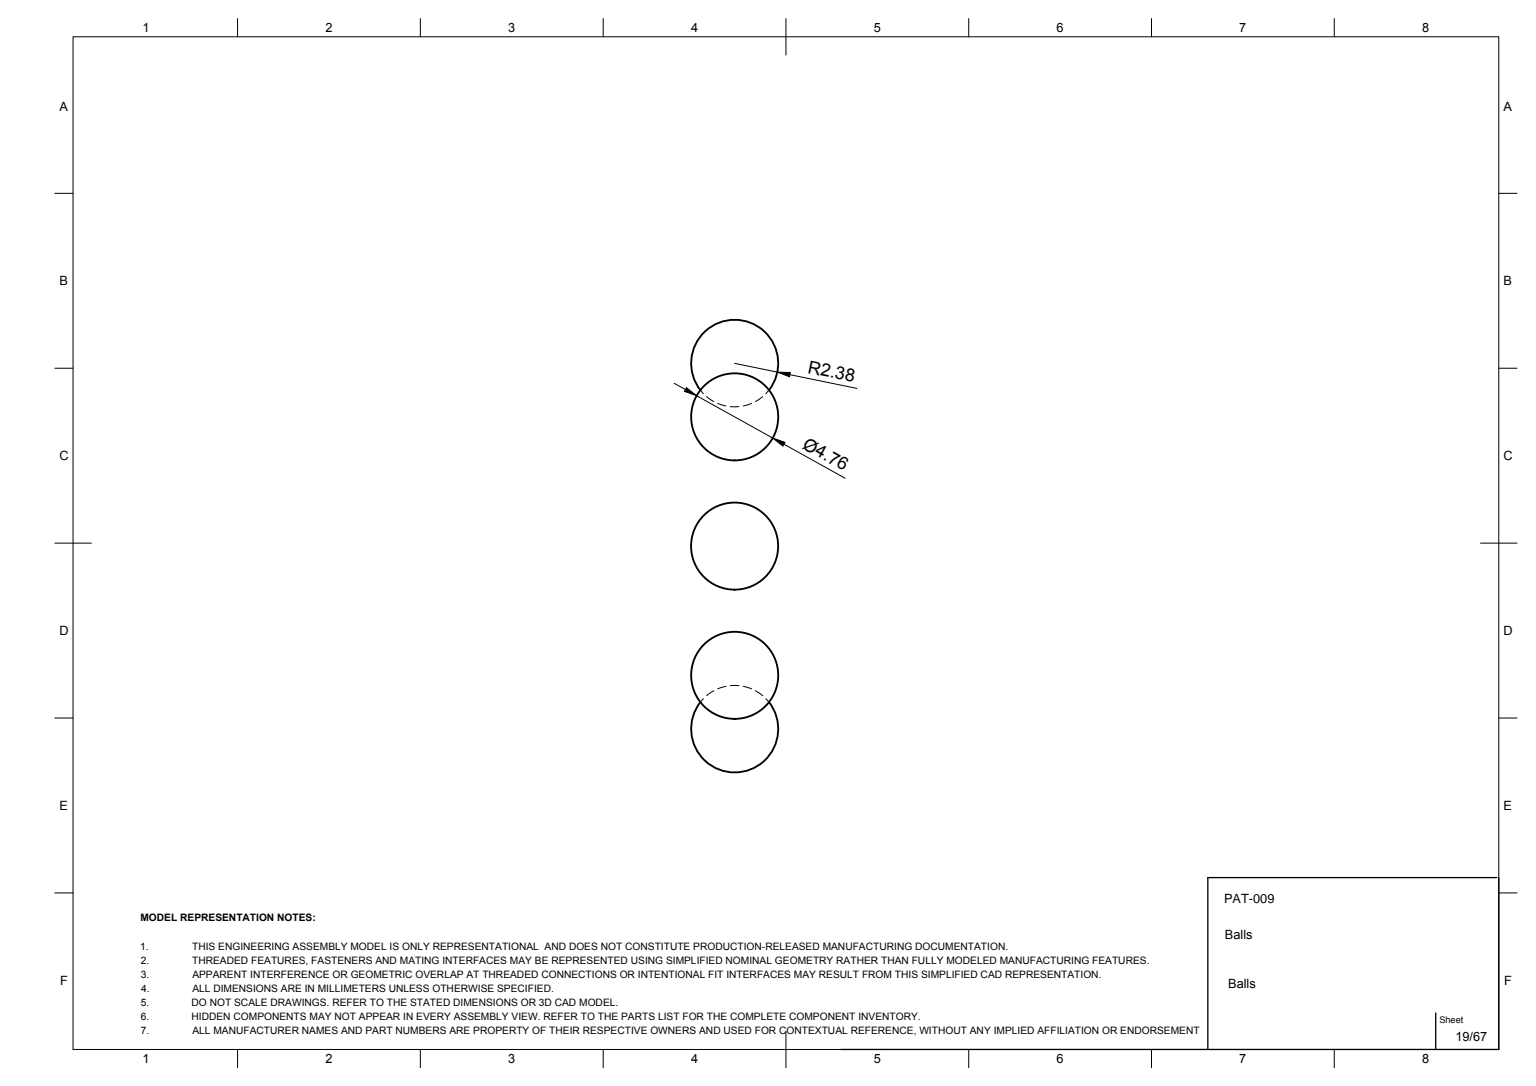
ISO-10303-21;
HEADER;
/* Generated by software containing ST-Developer
 * from STEP Tools, Inc. (www.steptools.com) 
 */

FILE_DESCRIPTION(
/* description */ ('Bell-crank linkage with push rods'),
/* implementation_level */ '2;1');

FILE_NAME(
/* name */ 'Balls.step',
/* time_stamp */ '2026-10-28T03:25:15-07:00',
/* author */ (''),
/* organization */ (''),
/* preprocessor_version */ 'ST-DEVELOPER v20.2',
/* originating_system */ 'Autodesk Translation Framework v15.17.0.0',
/* authorisation */ '');

FILE_SCHEMA (('AUTOMOTIVE_DESIGN { 1 0 10303 214 3 1 1 }'));
ENDSEC;

DATA;
#10=MECHANICAL_DESIGN_GEOMETRIC_PRESENTATION_REPRESENTATION('',(#616,#617,#618,#619,#620,#621,#622,#623),#16678);
#415=SPHERICAL_SURFACE('',#9830,0.23815);
#416=SPHERICAL_SURFACE('',#9832,0.23815);
#417=SPHERICAL_SURFACE('',#9834,0.23815);
#418=SPHERICAL_SURFACE('',#9836,0.23815);
#419=SPHERICAL_SURFACE('',#9838,0.23815);
#420=SPHERICAL_SURFACE('',#9840,0.23815);
#421=SPHERICAL_SURFACE('',#9842,0.23815);
#422=SPHERICAL_SURFACE('',#9844,0.23815);
#508=SHAPE_REPRESENTATION_RELATIONSHIP('SRR','None',#16925,#562);
#562=ADVANCED_BREP_SHAPE_REPRESENTATION('',(#677,#678,#679,#680,#681,#682,
#683,#684),#16630);
#616=STYLED_ITEM('',(#17291),#677);
#617=STYLED_ITEM('',(#17291),#678);
#618=STYLED_ITEM('',(#17291),#679);
#619=STYLED_ITEM('',(#17291),#680);
#620=STYLED_ITEM('',(#17291),#681);
#621=STYLED_ITEM('',(#17291),#682);
#622=STYLED_ITEM('',(#17291),#683);
#623=STYLED_ITEM('',(#17291),#684);
#677=MANIFOLD_SOLID_BREP('Body1',#8807);
#678=MANIFOLD_SOLID_BREP('Body2',#8808);
#679=MANIFOLD_SOLID_BREP('Body3',#8809);
#680=MANIFOLD_SOLID_BREP('Body4',#8810);
#681=MANIFOLD_SOLID_BREP('Body5',#8811);
#682=MANIFOLD_SOLID_BREP('Body6',#8812);
#683=MANIFOLD_SOLID_BREP('Body7',#8813);
#684=MANIFOLD_SOLID_BREP('Body8',#8814);
#1426=FACE_OUTER_BOUND('',#2040,.T.);
#1427=FACE_OUTER_BOUND('',#2041,.T.);
#1428=FACE_OUTER_BOUND('',#2042,.T.);
#1429=FACE_OUTER_BOUND('',#2043,.T.);
#1430=FACE_OUTER_BOUND('',#2044,.T.);
#1431=FACE_OUTER_BOUND('',#2045,.T.);
#1432=FACE_OUTER_BOUND('',#2046,.T.);
#1433=FACE_OUTER_BOUND('',#2047,.T.);
#2040=EDGE_LOOP('',(#6739,#6740));
#2041=EDGE_LOOP('',(#6741,#6742));
#2042=EDGE_LOOP('',(#6743,#6744));
#2043=EDGE_LOOP('',(#6745,#6746));
#2044=EDGE_LOOP('',(#6747,#6748));
#2045=EDGE_LOOP('',(#6749,#6750));
#2046=EDGE_LOOP('',(#6751,#6752));
#2047=EDGE_LOOP('',(#6753,#6754));
#3811=CIRCLE('',#9831,0.23815);
#3812=CIRCLE('',#9833,0.23815);
#3813=CIRCLE('',#9835,0.23815);
#3814=CIRCLE('',#9837,0.23815);
#3815=CIRCLE('',#9839,0.23815);
#3816=CIRCLE('',#9841,0.23815);
#3817=CIRCLE('',#9843,0.23815);
#3818=CIRCLE('',#9845,0.23815);
#4383=VERTEX_POINT('',#14548);
#4384=VERTEX_POINT('',#14549);
#4385=VERTEX_POINT('',#14552);
#4386=VERTEX_POINT('',#14553);
#4387=VERTEX_POINT('',#14556);
#4388=VERTEX_POINT('',#14557);
#4389=VERTEX_POINT('',#14560);
#4390=VERTEX_POINT('',#14561);
#4391=VERTEX_POINT('',#14564);
#4392=VERTEX_POINT('',#14565);
#4393=VERTEX_POINT('',#14568);
#4394=VERTEX_POINT('',#14569);
#4395=VERTEX_POINT('',#14572);
#4396=VERTEX_POINT('',#14573);
#4397=VERTEX_POINT('',#14576);
#4398=VERTEX_POINT('',#14577);
#5247=EDGE_CURVE('',#4383,#4384,#3811,.T.);
#5248=EDGE_CURVE('',#4385,#4386,#3812,.T.);
#5249=EDGE_CURVE('',#4387,#4388,#3813,.T.);
#5250=EDGE_CURVE('',#4389,#4390,#3814,.T.);
#5251=EDGE_CURVE('',#4391,#4392,#3815,.T.);
#5252=EDGE_CURVE('',#4393,#4394,#3816,.T.);
#5253=EDGE_CURVE('',#4395,#4396,#3817,.T.);
#5254=EDGE_CURVE('',#4397,#4398,#3818,.T.);
#6739=ORIENTED_EDGE('',*,*,#5247,.T.);
#6740=ORIENTED_EDGE('',*,*,#5247,.F.);
#6741=ORIENTED_EDGE('',*,*,#5248,.T.);
#6742=ORIENTED_EDGE('',*,*,#5248,.F.);
#6743=ORIENTED_EDGE('',*,*,#5249,.T.);
#6744=ORIENTED_EDGE('',*,*,#5249,.F.);
#6745=ORIENTED_EDGE('',*,*,#5250,.T.);
#6746=ORIENTED_EDGE('',*,*,#5250,.F.);
#6747=ORIENTED_EDGE('',*,*,#5251,.T.);
#6748=ORIENTED_EDGE('',*,*,#5251,.F.);
#6749=ORIENTED_EDGE('',*,*,#5252,.T.);
#6750=ORIENTED_EDGE('',*,*,#5252,.F.);
#6751=ORIENTED_EDGE('',*,*,#5253,.T.);
#6752=ORIENTED_EDGE('',*,*,#5253,.F.);
#6753=ORIENTED_EDGE('',*,*,#5254,.T.);
#6754=ORIENTED_EDGE('',*,*,#5254,.F.);
#8451=ADVANCED_FACE('',(#1426),#415,.T.);
#8452=ADVANCED_FACE('',(#1427),#416,.T.);
#8453=ADVANCED_FACE('',(#1428),#417,.T.);
#8454=ADVANCED_FACE('',(#1429),#418,.T.);
#8455=ADVANCED_FACE('',(#1430),#419,.T.);
#8456=ADVANCED_FACE('',(#1431),#420,.T.);
#8457=ADVANCED_FACE('',(#1432),#421,.T.);
#8458=ADVANCED_FACE('',(#1433),#422,.T.);
#8807=CLOSED_SHELL('',(#8451));
#8808=CLOSED_SHELL('',(#8452));
#8809=CLOSED_SHELL('',(#8453));
#8810=CLOSED_SHELL('',(#8454));
#8811=CLOSED_SHELL('',(#8455));
#8812=CLOSED_SHELL('',(#8456));
#8813=CLOSED_SHELL('',(#8457));
#8814=CLOSED_SHELL('',(#8458));
#9829=AXIS2_PLACEMENT_3D('',#14546,#11597,#11598);
#9830=AXIS2_PLACEMENT_3D('',#14547,#11599,#11600);
#9831=AXIS2_PLACEMENT_3D('',#14550,#11601,#11602);
#9832=AXIS2_PLACEMENT_3D('',#14551,#11603,#11604);
#9833=AXIS2_PLACEMENT_3D('',#14554,#11605,#11606);
#9834=AXIS2_PLACEMENT_3D('',#14555,#11607,#11608);
#9835=AXIS2_PLACEMENT_3D('',#14558,#11609,#11610);
#9836=AXIS2_PLACEMENT_3D('',#14559,#11611,#11612);
#9837=AXIS2_PLACEMENT_3D('',#14562,#11613,#11614);
#9838=AXIS2_PLACEMENT_3D('',#14563,#11615,#11616);
#9839=AXIS2_PLACEMENT_3D('',#14566,#11617,#11618);
#9840=AXIS2_PLACEMENT_3D('',#14567,#11619,#11620);
#9841=AXIS2_PLACEMENT_3D('',#14570,#11621,#11622);
#9842=AXIS2_PLACEMENT_3D('',#14571,#11623,#11624);
#9843=AXIS2_PLACEMENT_3D('',#14574,#11625,#11626);
#9844=AXIS2_PLACEMENT_3D('',#14575,#11627,#11628);
#9845=AXIS2_PLACEMENT_3D('',#14578,#11629,#11630);
#11597=DIRECTION('axis',(0.,0.,1.));
#11598=DIRECTION('refdir',(1.,0.,0.));
#11599=DIRECTION('center_axis',(0.,0.,1.));
#11600=DIRECTION('ref_axis',(1.,0.,0.));
#11601=DIRECTION('center_axis',(1.22464679914735E-16,-1.,0.));
#11602=DIRECTION('ref_axis',(-1.,-1.22464679914735E-16,0.));
#11603=DIRECTION('center_axis',(0.707106781186548,0.,0.707106781186548));
#11604=DIRECTION('ref_axis',(0.707106781186548,0.,-0.707106781186548));
#11605=DIRECTION('center_axis',(8.65956056235494E-17,-1.,-8.65956056235493E-17));
#11606=DIRECTION('ref_axis',(-0.707106781186547,-1.22464679914735E-16,0.707106781186547));
#11607=DIRECTION('center_axis',(1.,0.,0.));
#11608=DIRECTION('ref_axis',(6.12323399573676E-17,0.,-1.));
#11609=DIRECTION('center_axis',(7.49879891330929E-33,-1.,-1.22464679914735E-16));
#11610=DIRECTION('ref_axis',(-6.12323399573676E-17,-1.22464679914735E-16,
1.));
#11611=DIRECTION('center_axis',(0.707106781186548,0.,-0.707106781186548));
#11612=DIRECTION('ref_axis',(-0.707106781186548,0.,-0.707106781186548));
#11613=DIRECTION('center_axis',(-8.65956056235493E-17,-1.,-8.65956056235494E-17));
#11614=DIRECTION('ref_axis',(0.707106781186547,-1.22464679914735E-16,0.707106781186547));
#11615=DIRECTION('center_axis',(0.,0.,-1.));
#11616=DIRECTION('ref_axis',(-1.,0.,-1.22464679914735E-16));
#11617=DIRECTION('center_axis',(-1.22464679914735E-16,-1.,-1.49975978266186E-32));
#11618=DIRECTION('ref_axis',(1.,-1.22464679914735E-16,1.22464679914735E-16));
#11619=DIRECTION('center_axis',(-0.707106781186547,0.,-0.707106781186548));
#11620=DIRECTION('ref_axis',(-0.707106781186548,0.,0.707106781186547));
#11621=DIRECTION('center_axis',(-8.65956056235493E-17,-1.,8.65956056235493E-17));
#11622=DIRECTION('ref_axis',(0.707106781186548,-1.22464679914735E-16,-0.707106781186547));
#11623=DIRECTION('center_axis',(-1.,0.,0.));
#11624=DIRECTION('ref_axis',(-1.83697019872103E-16,0.,1.));
#11625=DIRECTION('center_axis',(-2.24963967399279E-32,-1.,1.22464679914735E-16));
#11626=DIRECTION('ref_axis',(1.83697019872103E-16,-1.22464679914735E-16,
-1.));
#11627=DIRECTION('center_axis',(-0.707106781186548,0.,0.707106781186548));
#11628=DIRECTION('ref_axis',(0.707106781186547,0.,0.707106781186548));
#11629=DIRECTION('center_axis',(8.65956056235493E-17,-1.,8.65956056235493E-17));
#11630=DIRECTION('ref_axis',(-0.707106781186547,-1.22464679914735E-16,-0.707106781186548));
#14546=CARTESIAN_POINT('',(0.,0.,0.));
#14547=CARTESIAN_POINT('Origin',(1.,0.,0.));
#14548=CARTESIAN_POINT('',(1.,-1.78583896120461E-33,0.23815));
#14549=CARTESIAN_POINT('',(1.,-1.78583896120461E-33,-0.23815));
#14550=CARTESIAN_POINT('Origin',(1.,0.,0.));
#14551=CARTESIAN_POINT('Origin',(0.707106781186548,0.,-0.707106781186547));
#14552=CARTESIAN_POINT('',(0.875504261126124,-1.78583896120461E-33,-0.538709301246971));
#14553=CARTESIAN_POINT('',(0.538709301246971,-1.78583896120461E-33,-0.875504261126124));
#14554=CARTESIAN_POINT('Origin',(0.707106781186548,0.,-0.707106781186547));
#14555=CARTESIAN_POINT('Origin',(6.12323399573677E-17,0.,-1.));
#14556=CARTESIAN_POINT('',(0.23815,-1.78583896120461E-33,-1.));
#14557=CARTESIAN_POINT('',(-0.23815,-1.78583896120461E-33,-1.));
#14558=CARTESIAN_POINT('Origin',(6.12323399573677E-17,0.,-1.));
#14559=CARTESIAN_POINT('Origin',(-0.707106781186547,0.,-0.707106781186548));
#14560=CARTESIAN_POINT('',(-0.538709301246971,-1.78583896120461E-33,-0.875504261126124));
#14561=CARTESIAN_POINT('',(-0.875504261126124,-1.78583896120461E-33,-0.538709301246971));
#14562=CARTESIAN_POINT('Origin',(-0.707106781186547,0.,-0.707106781186548));
#14563=CARTESIAN_POINT('Origin',(-1.,0.,-1.22464679914735E-16));
#14564=CARTESIAN_POINT('',(-1.,-1.78583896120461E-33,-0.23815));
#14565=CARTESIAN_POINT('',(-1.,-1.78583896120461E-33,0.23815));
#14566=CARTESIAN_POINT('Origin',(-1.,0.,-1.22464679914735E-16));
#14567=CARTESIAN_POINT('Origin',(-0.707106781186548,0.,0.707106781186547));
#14568=CARTESIAN_POINT('',(-0.875504261126124,-7.94881478324376E-33,0.538709301246971));
#14569=CARTESIAN_POINT('',(-0.538709301246971,4.37713686083455E-33,0.875504261126124));
#14570=CARTESIAN_POINT('Origin',(-0.707106781186548,0.,0.707106781186547));
#14571=CARTESIAN_POINT('Origin',(-1.83697019872103E-16,0.,1.));
#14572=CARTESIAN_POINT('',(-0.23815,-1.78583896120461E-33,1.));
#14573=CARTESIAN_POINT('',(0.23815,-1.78583896120461E-33,1.));
#14574=CARTESIAN_POINT('Origin',(-1.83697019872103E-16,0.,1.));
#14575=CARTESIAN_POINT('Origin',(0.707106781186547,0.,0.707106781186548));
#14576=CARTESIAN_POINT('',(0.538709301246971,-4.86732687222419E-33,0.875504261126124));
#14577=CARTESIAN_POINT('',(0.875504261126124,1.29564894981497E-33,0.538709301246971));
#14578=CARTESIAN_POINT('Origin',(0.707106781186547,0.,0.707106781186548));
#16566=UNCERTAINTY_MEASURE_WITH_UNIT(LENGTH_MEASURE(0.001),#16679,
'DISTANCE_ACCURACY_VALUE',
'Maximum model space distance between geometric entities at asserted c
onnectivities');
#16614=UNCERTAINTY_MEASURE_WITH_UNIT(LENGTH_MEASURE(0.001),#16679,
'DISTANCE_ACCURACY_VALUE',
'Maximum model space distance between geometric entities at asserted c
onnectivities');
#16630=(
GEOMETRIC_REPRESENTATION_CONTEXT(3)
GLOBAL_UNCERTAINTY_ASSIGNED_CONTEXT((#16566))
GLOBAL_UNIT_ASSIGNED_CONTEXT((#16679,#16681,#16682))
REPRESENTATION_CONTEXT('','3D')
);
#16678=(
GEOMETRIC_REPRESENTATION_CONTEXT(3)
GLOBAL_UNCERTAINTY_ASSIGNED_CONTEXT((#16614))
GLOBAL_UNIT_ASSIGNED_CONTEXT((#16679,#16681,#16682))
REPRESENTATION_CONTEXT('','3D')
);
#16679=(
LENGTH_UNIT()
NAMED_UNIT(*)
SI_UNIT(.CENTI.,.METRE.)
);
#16681=(
NAMED_UNIT(*)
PLANE_ANGLE_UNIT()
SI_UNIT($,.RADIAN.)
);
#16682=(
NAMED_UNIT(*)
SI_UNIT($,.STERADIAN.)
SOLID_ANGLE_UNIT()
);
#16698=SHAPE_DEFINITION_REPRESENTATION(#16761,#16925);
#16761=PRODUCT_DEFINITION_SHAPE('',$,#16989);
#16925=SHAPE_REPRESENTATION('',(#9829),#16630);
#16973=PRODUCT_DEFINITION_CONTEXT('part definition',#17164,'design');
#16989=PRODUCT_DEFINITION('Balls','Balls',#17052,#16973);
#17052=PRODUCT_DEFINITION_FORMATION('',$,#17181);
#17164=APPLICATION_CONTEXT(
'Core Data for Automotive Mechanical Design Process');
#17165=PRODUCT_CONTEXT('part definition',#17164,'mechanical');
#17181=PRODUCT('Balls','Balls','Balls',(#17165));
#17285=COLOUR_RGB('Grey',0.48,0.52,0.57);
#17286=FILL_AREA_STYLE_COLOUR('',#17285);
#17287=FILL_AREA_STYLE('',(#17286));
#17288=SURFACE_STYLE_FILL_AREA(#17287);
#17289=SURFACE_SIDE_STYLE('',(#17288));
#17290=SURFACE_STYLE_USAGE(.BOTH.,#17289);
#17291=PRESENTATION_STYLE_ASSIGNMENT((#17290));
ENDSEC;
END-ISO-10303-21;
